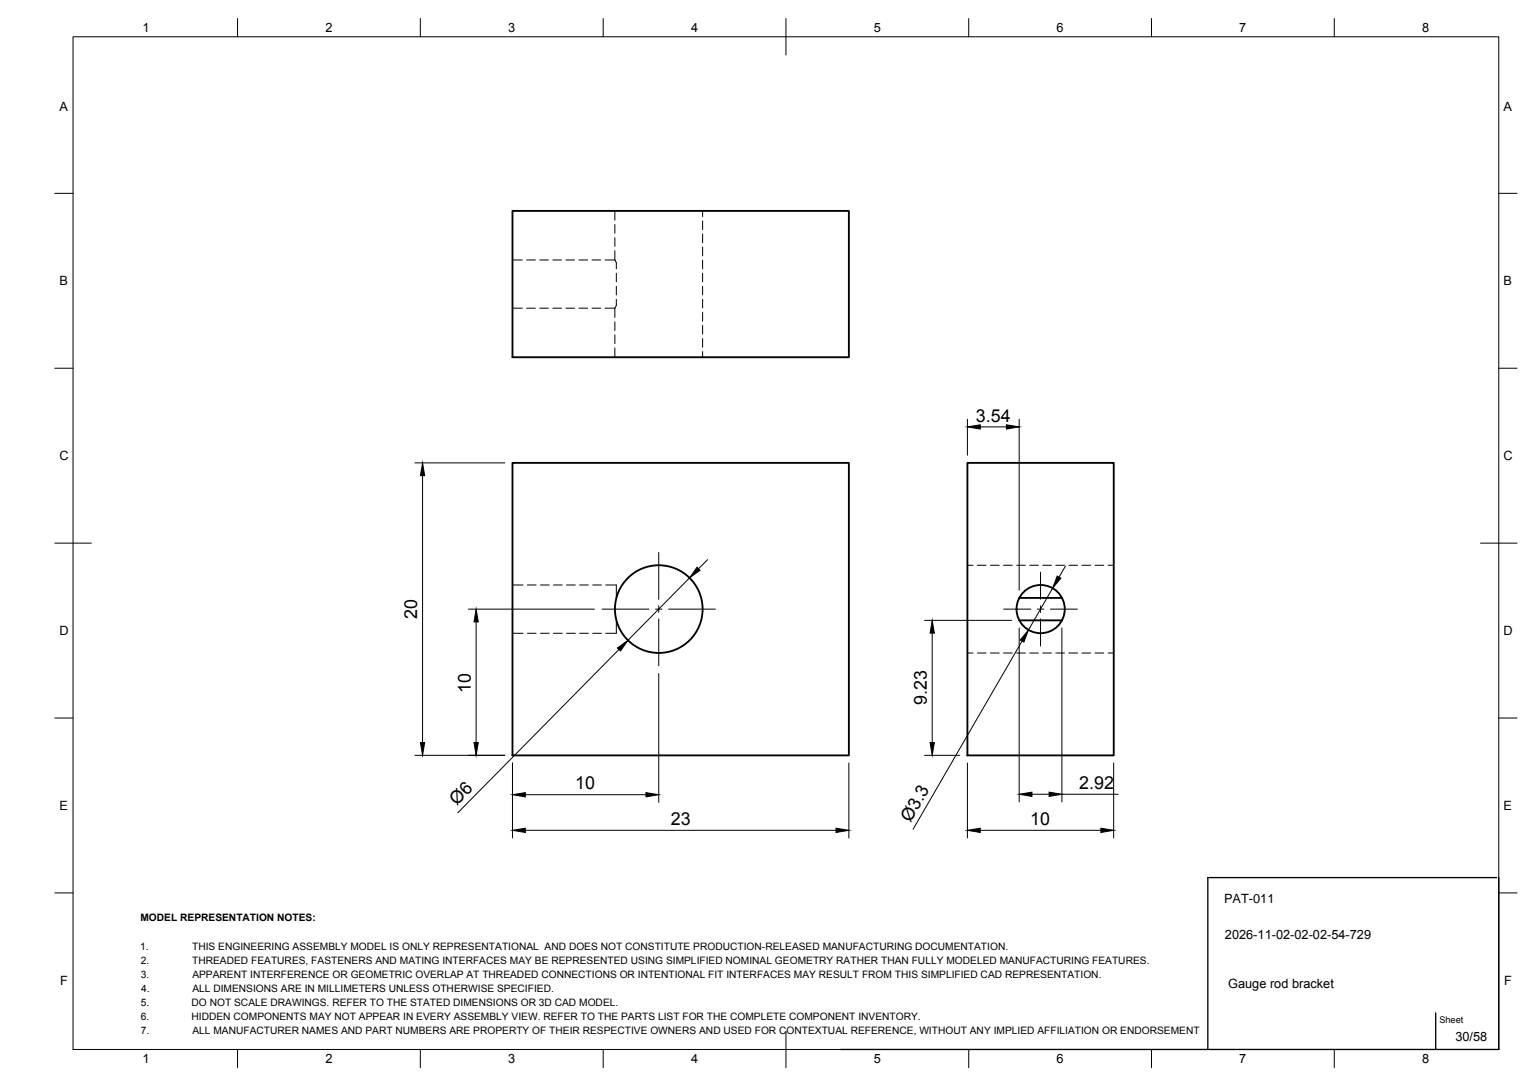
ISO-10303-21;
HEADER;
/* Generated by software containing ST-Developer
 * from STEP Tools, Inc. (www.steptools.com) 
 */

FILE_DESCRIPTION(
/* description */ ('Belt tension measurement rig'),
/* implementation_level */ '2;1');

FILE_NAME(
/* name */ 'Gauge rod bracket.step',
/* time_stamp */ '2026-10-28T03:24:44-07:00',
/* author */ (''),
/* organization */ (''),
/* preprocessor_version */ 'ST-DEVELOPER v20.2',
/* originating_system */ 'Autodesk Translation Framework v15.17.0.0',
/* authorisation */ '');

FILE_SCHEMA (('AUTOMOTIVE_DESIGN { 1 0 10303 214 3 1 1 }'));
ENDSEC;

DATA;
#10=MECHANICAL_DESIGN_GEOMETRIC_PRESENTATION_REPRESENTATION('',(#726),#23587);
#513=B_SPLINE_CURVE_WITH_KNOTS('',3,(#20469,#20470,#20471,#20472,#20473,
#20474),.UNSPECIFIED.,.F.,.F.,(4,2,4),(0.687371506923446,0.701311490231616,
0.764919212052549),.UNSPECIFIED.);
#514=B_SPLINE_CURVE_WITH_KNOTS('',3,(#20478,#20479,#20480,#20481,#20482,
#20483),.UNSPECIFIED.,.F.,.F.,(4,2,4),(0.254973070684183,0.318580792505116,
0.332520775813288),.UNSPECIFIED.);
#515=B_SPLINE_CURVE_WITH_KNOTS('',3,(#20484,#20485,#20486,#20487,#20488,
#20489),.UNSPECIFIED.,.F.,.F.,(4,2,4),(0.177425365555078,0.19136534886325,
0.254973070684183),.UNSPECIFIED.);
#516=B_SPLINE_CURVE_WITH_KNOTS('',3,(#20490,#20491,#20492,#20493,#20494,
#20495),.UNSPECIFIED.,.F.,.F.,(4,2,4),(0.764919212052549,0.828526933873482,
0.842466917181652),.UNSPECIFIED.);
#608=SHAPE_REPRESENTATION_RELATIONSHIP('SRR','None',#23855,#663);
#663=ADVANCED_BREP_SHAPE_REPRESENTATION('',(#796),#23553);
#726=STYLED_ITEM('',(#24211),#796);
#796=MANIFOLD_SOLID_BREP('Body1',#12231);
#966=FACE_BOUND('',#2514,.T.);
#967=FACE_BOUND('',#2517,.T.);
#968=FACE_BOUND('',#2519,.T.);
#1193=PLANE('',#13549);
#1194=PLANE('',#13554);
#1195=PLANE('',#13558);
#1196=PLANE('',#13559);
#1197=PLANE('',#13560);
#1198=PLANE('',#13561);
#1199=PLANE('',#13562);
#1200=PLANE('',#13563);
#1667=FACE_OUTER_BOUND('',#2508,.T.);
#1668=FACE_OUTER_BOUND('',#2509,.T.);
#1669=FACE_OUTER_BOUND('',#2510,.T.);
#1670=FACE_OUTER_BOUND('',#2511,.T.);
#1671=FACE_OUTER_BOUND('',#2512,.T.);
#1672=FACE_OUTER_BOUND('',#2513,.T.);
#1673=FACE_OUTER_BOUND('',#2515,.T.);
#1674=FACE_OUTER_BOUND('',#2516,.T.);
#1675=FACE_OUTER_BOUND('',#2518,.T.);
#1676=FACE_OUTER_BOUND('',#2520,.T.);
#2508=EDGE_LOOP('',(#9310,#9311));
#2509=EDGE_LOOP('',(#9312,#9313,#9314,#9315,#9316,#9317,#9318,#9319,#9320));
#2510=EDGE_LOOP('',(#9321,#9322));
#2511=EDGE_LOOP('',(#9323,#9324,#9325,#9326,#9327,#9328,#9329,#9330,#9331,
#9332,#9333,#9334));
#2512=EDGE_LOOP('',(#9335,#9336,#9337,#9338));
#2513=EDGE_LOOP('',(#9339,#9340,#9341,#9342));
#2514=EDGE_LOOP('',(#9343));
#2515=EDGE_LOOP('',(#9344,#9345,#9346,#9347));
#2516=EDGE_LOOP('',(#9348,#9349,#9350,#9351));
#2517=EDGE_LOOP('',(#9352));
#2518=EDGE_LOOP('',(#9353,#9354,#9355,#9356));
#2519=EDGE_LOOP('',(#9357));
#2520=EDGE_LOOP('',(#9358,#9359,#9360,#9361));
#3310=LINE('',#20464,#4061);
#3311=LINE('',#20497,#4062);
#3312=LINE('',#20500,#4063);
#3313=LINE('',#20504,#4064);
#3314=LINE('',#20506,#4065);
#3315=LINE('',#20511,#4066);
#3316=LINE('',#20513,#4067);
#3317=LINE('',#20515,#4068);
#3318=LINE('',#20516,#4069);
#3319=LINE('',#20519,#4070);
#3320=LINE('',#20521,#4071);
#3321=LINE('',#20522,#4072);
#3322=LINE('',#20525,#4073);
#3323=LINE('',#20527,#4074);
#3324=LINE('',#20528,#4075);
#3325=LINE('',#20530,#4076);
#3326=LINE('',#20531,#4077);
#4061=VECTOR('',#16207,1.);
#4062=VECTOR('',#16214,0.164999999999999);
#4063=VECTOR('',#16219,1.);
#4064=VECTOR('',#16224,0.3);
#4065=VECTOR('',#16225,0.3);
#4066=VECTOR('',#16230,1.);
#4067=VECTOR('',#16231,1.);
#4068=VECTOR('',#16232,1.);
#4069=VECTOR('',#16233,1.);
#4070=VECTOR('',#16236,1.);
#4071=VECTOR('',#16237,1.);
#4072=VECTOR('',#16238,1.);
#4073=VECTOR('',#16241,1.);
#4074=VECTOR('',#16242,1.);
#4075=VECTOR('',#16243,1.);
#4076=VECTOR('',#16246,1.);
#4077=VECTOR('',#16247,1.);
#4792=CIRCLE('',#13550,0.164999999999999);
#4793=CIRCLE('',#13552,0.164999999999999);
#4794=CIRCLE('',#13553,0.164999999999999);
#4795=CIRCLE('',#13556,0.3);
#4796=CIRCLE('',#13557,0.3);
#5702=VERTEX_POINT('',#20462);
#5703=VERTEX_POINT('',#20463);
#5704=VERTEX_POINT('',#20467);
#5705=VERTEX_POINT('',#20468);
#5706=VERTEX_POINT('',#20475);
#5707=VERTEX_POINT('',#20477);
#5708=VERTEX_POINT('',#20496);
#5709=VERTEX_POINT('',#20502);
#5710=VERTEX_POINT('',#20505);
#5711=VERTEX_POINT('',#20509);
#5712=VERTEX_POINT('',#20510);
#5713=VERTEX_POINT('',#20512);
#5714=VERTEX_POINT('',#20514);
#5715=VERTEX_POINT('',#20518);
#5716=VERTEX_POINT('',#20520);
#5717=VERTEX_POINT('',#20524);
#5718=VERTEX_POINT('',#20526);
#7014=EDGE_CURVE('',#5702,#5703,#3310,.T.);
#7015=EDGE_CURVE('',#5702,#5703,#4792,.T.);
#7016=EDGE_CURVE('',#5704,#5705,#513,.T.);
#7017=EDGE_CURVE('',#5706,#5704,#4793,.T.);
#7018=EDGE_CURVE('',#5707,#5706,#514,.T.);
#7019=EDGE_CURVE('',#5703,#5707,#515,.T.);
#7020=EDGE_CURVE('',#5705,#5702,#516,.T.);
#7021=EDGE_CURVE('',#5705,#5708,#3311,.T.);
#7022=EDGE_CURVE('',#5708,#5708,#4794,.T.);
#7023=EDGE_CURVE('',#5706,#5704,#3312,.T.);
#7024=EDGE_CURVE('',#5709,#5709,#4795,.T.);
#7025=EDGE_CURVE('',#5709,#5705,#3313,.T.);
#7026=EDGE_CURVE('',#5707,#5710,#3314,.T.);
#7027=EDGE_CURVE('',#5710,#5710,#4796,.T.);
#7028=EDGE_CURVE('',#5711,#5712,#3315,.T.);
#7029=EDGE_CURVE('',#5712,#5713,#3316,.T.);
#7030=EDGE_CURVE('',#5714,#5713,#3317,.T.);
#7031=EDGE_CURVE('',#5711,#5714,#3318,.T.);
#7032=EDGE_CURVE('',#5715,#5711,#3319,.T.);
#7033=EDGE_CURVE('',#5716,#5714,#3320,.T.);
#7034=EDGE_CURVE('',#5715,#5716,#3321,.T.);
#7035=EDGE_CURVE('',#5717,#5715,#3322,.T.);
#7036=EDGE_CURVE('',#5718,#5716,#3323,.T.);
#7037=EDGE_CURVE('',#5717,#5718,#3324,.T.);
#7038=EDGE_CURVE('',#5712,#5717,#3325,.T.);
#7039=EDGE_CURVE('',#5713,#5718,#3326,.T.);
#9310=ORIENTED_EDGE('',*,*,#7014,.F.);
#9311=ORIENTED_EDGE('',*,*,#7015,.T.);
#9312=ORIENTED_EDGE('',*,*,#7016,.F.);
#9313=ORIENTED_EDGE('',*,*,#7017,.F.);
#9314=ORIENTED_EDGE('',*,*,#7018,.F.);
#9315=ORIENTED_EDGE('',*,*,#7019,.F.);
#9316=ORIENTED_EDGE('',*,*,#7015,.F.);
#9317=ORIENTED_EDGE('',*,*,#7020,.F.);
#9318=ORIENTED_EDGE('',*,*,#7021,.T.);
#9319=ORIENTED_EDGE('',*,*,#7022,.F.);
#9320=ORIENTED_EDGE('',*,*,#7021,.F.);
#9321=ORIENTED_EDGE('',*,*,#7023,.F.);
#9322=ORIENTED_EDGE('',*,*,#7017,.T.);
#9323=ORIENTED_EDGE('',*,*,#7024,.F.);
#9324=ORIENTED_EDGE('',*,*,#7025,.T.);
#9325=ORIENTED_EDGE('',*,*,#7020,.T.);
#9326=ORIENTED_EDGE('',*,*,#7014,.T.);
#9327=ORIENTED_EDGE('',*,*,#7019,.T.);
#9328=ORIENTED_EDGE('',*,*,#7026,.T.);
#9329=ORIENTED_EDGE('',*,*,#7027,.F.);
#9330=ORIENTED_EDGE('',*,*,#7026,.F.);
#9331=ORIENTED_EDGE('',*,*,#7018,.T.);
#9332=ORIENTED_EDGE('',*,*,#7023,.T.);
#9333=ORIENTED_EDGE('',*,*,#7016,.T.);
#9334=ORIENTED_EDGE('',*,*,#7025,.F.);
#9335=ORIENTED_EDGE('',*,*,#7028,.T.);
#9336=ORIENTED_EDGE('',*,*,#7029,.T.);
#9337=ORIENTED_EDGE('',*,*,#7030,.F.);
#9338=ORIENTED_EDGE('',*,*,#7031,.F.);
#9339=ORIENTED_EDGE('',*,*,#7032,.T.);
#9340=ORIENTED_EDGE('',*,*,#7031,.T.);
#9341=ORIENTED_EDGE('',*,*,#7033,.F.);
#9342=ORIENTED_EDGE('',*,*,#7034,.F.);
#9343=ORIENTED_EDGE('',*,*,#7027,.T.);
#9344=ORIENTED_EDGE('',*,*,#7035,.T.);
#9345=ORIENTED_EDGE('',*,*,#7034,.T.);
#9346=ORIENTED_EDGE('',*,*,#7036,.F.);
#9347=ORIENTED_EDGE('',*,*,#7037,.F.);
#9348=ORIENTED_EDGE('',*,*,#7038,.T.);
#9349=ORIENTED_EDGE('',*,*,#7037,.T.);
#9350=ORIENTED_EDGE('',*,*,#7039,.F.);
#9351=ORIENTED_EDGE('',*,*,#7029,.F.);
#9352=ORIENTED_EDGE('',*,*,#7024,.T.);
#9353=ORIENTED_EDGE('',*,*,#7039,.T.);
#9354=ORIENTED_EDGE('',*,*,#7036,.T.);
#9355=ORIENTED_EDGE('',*,*,#7033,.T.);
#9356=ORIENTED_EDGE('',*,*,#7030,.T.);
#9357=ORIENTED_EDGE('',*,*,#7022,.T.);
#9358=ORIENTED_EDGE('',*,*,#7038,.F.);
#9359=ORIENTED_EDGE('',*,*,#7028,.F.);
#9360=ORIENTED_EDGE('',*,*,#7032,.F.);
#9361=ORIENTED_EDGE('',*,*,#7035,.F.);
#11295=CYLINDRICAL_SURFACE('',#13551,0.164999999999999);
#11296=CYLINDRICAL_SURFACE('',#13555,0.3);
#11808=ADVANCED_FACE('',(#1667),#1193,.T.);
#11809=ADVANCED_FACE('',(#1668),#11295,.F.);
#11810=ADVANCED_FACE('',(#1669),#1194,.T.);
#11811=ADVANCED_FACE('',(#1670),#11296,.F.);
#11812=ADVANCED_FACE('',(#1671),#1195,.T.);
#11813=ADVANCED_FACE('',(#1672,#966),#1196,.T.);
#11814=ADVANCED_FACE('',(#1673),#1197,.T.);
#11815=ADVANCED_FACE('',(#1674,#967),#1198,.T.);
#11816=ADVANCED_FACE('',(#1675,#968),#1199,.T.);
#11817=ADVANCED_FACE('',(#1676),#1200,.F.);
#12231=CLOSED_SHELL('',(#11808,#11809,#11810,#11811,#11812,#11813,#11814,
#11815,#11816,#11817));
#13548=AXIS2_PLACEMENT_3D('',#20460,#16203,#16204);
#13549=AXIS2_PLACEMENT_3D('',#20461,#16205,#16206);
#13550=AXIS2_PLACEMENT_3D('',#20465,#16208,#16209);
#13551=AXIS2_PLACEMENT_3D('',#20466,#16210,#16211);
#13552=AXIS2_PLACEMENT_3D('',#20476,#16212,#16213);
#13553=AXIS2_PLACEMENT_3D('',#20498,#16215,#16216);
#13554=AXIS2_PLACEMENT_3D('',#20499,#16217,#16218);
#13555=AXIS2_PLACEMENT_3D('',#20501,#16220,#16221);
#13556=AXIS2_PLACEMENT_3D('',#20503,#16222,#16223);
#13557=AXIS2_PLACEMENT_3D('',#20507,#16226,#16227);
#13558=AXIS2_PLACEMENT_3D('',#20508,#16228,#16229);
#13559=AXIS2_PLACEMENT_3D('',#20517,#16234,#16235);
#13560=AXIS2_PLACEMENT_3D('',#20523,#16239,#16240);
#13561=AXIS2_PLACEMENT_3D('',#20529,#16244,#16245);
#13562=AXIS2_PLACEMENT_3D('',#20532,#16248,#16249);
#13563=AXIS2_PLACEMENT_3D('',#20533,#16250,#16251);
#16203=DIRECTION('axis',(0.,0.,1.));
#16204=DIRECTION('refdir',(1.,0.,0.));
#16205=DIRECTION('center_axis',(0.,0.,1.));
#16206=DIRECTION('ref_axis',(1.,0.,0.));
#16207=DIRECTION('',(1.,0.,0.));
#16208=DIRECTION('center_axis',(0.,0.,1.));
#16209=DIRECTION('ref_axis',(1.,0.,0.));
#16210=DIRECTION('center_axis',(0.,0.,1.));
#16211=DIRECTION('ref_axis',(1.,0.,0.));
#16212=DIRECTION('center_axis',(0.,0.,1.));
#16213=DIRECTION('ref_axis',(1.,0.,0.));
#16214=DIRECTION('',(0.,0.,1.));
#16215=DIRECTION('center_axis',(0.,0.,-1.));
#16216=DIRECTION('ref_axis',(1.,0.,0.));
#16217=DIRECTION('center_axis',(0.,0.,1.));
#16218=DIRECTION('ref_axis',(1.,0.,0.));
#16219=DIRECTION('',(-1.,0.,0.));
#16220=DIRECTION('center_axis',(1.,0.,0.));
#16221=DIRECTION('ref_axis',(0.,0.,-1.));
#16222=DIRECTION('center_axis',(1.,0.,0.));
#16223=DIRECTION('ref_axis',(0.,0.,-1.));
#16224=DIRECTION('',(1.,0.,0.));
#16225=DIRECTION('',(1.,0.,0.));
#16226=DIRECTION('center_axis',(-1.,0.,0.));
#16227=DIRECTION('ref_axis',(0.,0.,-1.));
#16228=DIRECTION('center_axis',(0.,1.,0.));
#16229=DIRECTION('ref_axis',(-1.,0.,0.));
#16230=DIRECTION('',(-1.,0.,0.));
#16231=DIRECTION('',(0.,0.,1.));
#16232=DIRECTION('',(-1.,0.,0.));
#16233=DIRECTION('',(0.,0.,1.));
#16234=DIRECTION('center_axis',(1.,0.,0.));
#16235=DIRECTION('ref_axis',(0.,1.,0.));
#16236=DIRECTION('',(0.,1.,0.));
#16237=DIRECTION('',(0.,1.,0.));
#16238=DIRECTION('',(0.,0.,1.));
#16239=DIRECTION('center_axis',(0.,-1.,0.));
#16240=DIRECTION('ref_axis',(1.,0.,0.));
#16241=DIRECTION('',(1.,0.,0.));
#16242=DIRECTION('',(1.,0.,0.));
#16243=DIRECTION('',(0.,0.,1.));
#16244=DIRECTION('center_axis',(-1.,0.,0.));
#16245=DIRECTION('ref_axis',(0.,-1.,0.));
#16246=DIRECTION('',(0.,-1.,0.));
#16247=DIRECTION('',(0.,-1.,0.));
#16248=DIRECTION('center_axis',(0.,0.,1.));
#16249=DIRECTION('ref_axis',(1.,0.,0.));
#16250=DIRECTION('center_axis',(0.,0.,1.));
#16251=DIRECTION('ref_axis',(1.,0.,0.));
#20460=CARTESIAN_POINT('',(0.,0.,0.));
#20461=CARTESIAN_POINT('Origin',(13.5,7.5,4.79));
#20462=CARTESIAN_POINT('',(13.3539691813349,7.42318854252131,4.79));
#20463=CARTESIAN_POINT('',(13.6460308186651,7.42318854252131,4.79));
#20464=CARTESIAN_POINT('',(12.9,7.42318854252131,4.79));
#20465=CARTESIAN_POINT('Origin',(13.5,7.5,4.79));
#20466=CARTESIAN_POINT('Origin',(13.5,7.5,4.79));
#20467=CARTESIAN_POINT('',(13.3539691813349,7.57681145747869,4.79));
#20468=CARTESIAN_POINT('',(13.335,7.5,4.8));
#20469=CARTESIAN_POINT('Ctrl Pts',(13.3539691813349,7.57681145747868,4.79));
#20470=CARTESIAN_POINT('Ctrl Pts',(13.3517424038809,7.57257799875687,4.79112130391241));
#20471=CARTESIAN_POINT('Ctrl Pts',(13.3496896532208,7.56822754447862,4.79217403693718));
#20472=CARTESIAN_POINT('Ctrl Pts',(13.3393317115009,7.54351674734392,4.79755094970157));
#20473=CARTESIAN_POINT('Ctrl Pts',(13.335,7.52120257394031,4.8));
#20474=CARTESIAN_POINT('Ctrl Pts',(13.335,7.5,4.8));
#20475=CARTESIAN_POINT('',(13.6460308186651,7.57681145747869,4.79));
#20476=CARTESIAN_POINT('Origin',(13.5,7.5,4.79));
#20477=CARTESIAN_POINT('',(13.665,7.5,4.8));
#20478=CARTESIAN_POINT('Ctrl Pts',(13.665,7.5,4.8));
#20479=CARTESIAN_POINT('Ctrl Pts',(13.665,7.52120257394031,4.8));
#20480=CARTESIAN_POINT('Ctrl Pts',(13.6606682884991,7.54351674734392,4.79755094970157));
#20481=CARTESIAN_POINT('Ctrl Pts',(13.6503103467792,7.56822754447862,4.79217403693718));
#20482=CARTESIAN_POINT('Ctrl Pts',(13.6482575961191,7.57257799875688,4.79112130391241));
#20483=CARTESIAN_POINT('Ctrl Pts',(13.6460308186651,7.57681145747869,4.79));
#20484=CARTESIAN_POINT('Ctrl Pts',(13.6460308186651,7.42318854252131,4.79));
#20485=CARTESIAN_POINT('Ctrl Pts',(13.6482575961191,7.42742200124312,4.79112130391241));
#20486=CARTESIAN_POINT('Ctrl Pts',(13.6503103467792,7.43177245552138,4.79217403693718));
#20487=CARTESIAN_POINT('Ctrl Pts',(13.6606682884991,7.45648325265608,4.79755094970157));
#20488=CARTESIAN_POINT('Ctrl Pts',(13.665,7.47879742605969,4.8));
#20489=CARTESIAN_POINT('Ctrl Pts',(13.665,7.5,4.8));
#20490=CARTESIAN_POINT('Ctrl Pts',(13.335,7.5,4.8));
#20491=CARTESIAN_POINT('Ctrl Pts',(13.335,7.47879742605969,4.8));
#20492=CARTESIAN_POINT('Ctrl Pts',(13.3393317115009,7.45648325265608,4.79755094970157));
#20493=CARTESIAN_POINT('Ctrl Pts',(13.3496896532208,7.43177245552138,4.79217403693718));
#20494=CARTESIAN_POINT('Ctrl Pts',(13.3517424038809,7.42742200124312,4.79112130391241));
#20495=CARTESIAN_POINT('Ctrl Pts',(13.3539691813349,7.42318854252132,4.79));
#20496=CARTESIAN_POINT('',(13.335,7.5,5.5));
#20497=CARTESIAN_POINT('',(13.335,7.5,4.79));
#20498=CARTESIAN_POINT('Origin',(13.5,7.5,5.5));
#20499=CARTESIAN_POINT('Origin',(13.5,7.5,4.79));
#20500=CARTESIAN_POINT('',(12.9,7.57681145747869,4.79));
#20501=CARTESIAN_POINT('Origin',(12.9,7.5,4.5));
#20502=CARTESIAN_POINT('',(13.,7.5,4.8));
#20503=CARTESIAN_POINT('Origin',(13.,7.5,4.5));
#20504=CARTESIAN_POINT('',(12.9,7.5,4.8));
#20505=CARTESIAN_POINT('',(14.,7.5,4.8));
#20506=CARTESIAN_POINT('',(12.9,7.5,4.8));
#20507=CARTESIAN_POINT('Origin',(14.,7.5,4.5));
#20508=CARTESIAN_POINT('Origin',(14.,8.5,3.2));
#20509=CARTESIAN_POINT('',(14.,8.5,3.2));
#20510=CARTESIAN_POINT('',(13.,8.5,3.2));
#20511=CARTESIAN_POINT('',(14.,8.5,3.2));
#20512=CARTESIAN_POINT('',(13.,8.5,5.5));
#20513=CARTESIAN_POINT('',(13.,8.5,3.2));
#20514=CARTESIAN_POINT('',(14.,8.5,5.5));
#20515=CARTESIAN_POINT('',(14.,8.5,5.5));
#20516=CARTESIAN_POINT('',(14.,8.5,3.2));
#20517=CARTESIAN_POINT('Origin',(14.,6.5,3.2));
#20518=CARTESIAN_POINT('',(14.,6.5,3.2));
#20519=CARTESIAN_POINT('',(14.,6.5,3.2));
#20520=CARTESIAN_POINT('',(14.,6.5,5.5));
#20521=CARTESIAN_POINT('',(14.,6.5,5.5));
#20522=CARTESIAN_POINT('',(14.,6.5,3.2));
#20523=CARTESIAN_POINT('Origin',(13.,6.5,3.2));
#20524=CARTESIAN_POINT('',(13.,6.5,3.2));
#20525=CARTESIAN_POINT('',(13.,6.5,3.2));
#20526=CARTESIAN_POINT('',(13.,6.5,5.5));
#20527=CARTESIAN_POINT('',(13.,6.5,5.5));
#20528=CARTESIAN_POINT('',(13.,6.5,3.2));
#20529=CARTESIAN_POINT('Origin',(13.,8.5,3.2));
#20530=CARTESIAN_POINT('',(13.,8.5,3.2));
#20531=CARTESIAN_POINT('',(13.,8.5,5.5));
#20532=CARTESIAN_POINT('Origin',(13.5,7.5,5.5));
#20533=CARTESIAN_POINT('Origin',(13.5,7.5,3.2));
#23488=UNCERTAINTY_MEASURE_WITH_UNIT(LENGTH_MEASURE(0.001),#23588,
'DISTANCE_ACCURACY_VALUE',
'Maximum model space distance between geometric entities at asserted c
onnectivities');
#23522=UNCERTAINTY_MEASURE_WITH_UNIT(LENGTH_MEASURE(0.001),#23588,
'DISTANCE_ACCURACY_VALUE',
'Maximum model space distance between geometric entities at asserted c
onnectivities');
#23553=(
GEOMETRIC_REPRESENTATION_CONTEXT(3)
GLOBAL_UNCERTAINTY_ASSIGNED_CONTEXT((#23488))
GLOBAL_UNIT_ASSIGNED_CONTEXT((#23588,#23590,#23591))
REPRESENTATION_CONTEXT('','3D')
);
#23587=(
GEOMETRIC_REPRESENTATION_CONTEXT(3)
GLOBAL_UNCERTAINTY_ASSIGNED_CONTEXT((#23522))
GLOBAL_UNIT_ASSIGNED_CONTEXT((#23588,#23590,#23591))
REPRESENTATION_CONTEXT('','3D')
);
#23588=(
LENGTH_UNIT()
NAMED_UNIT(*)
SI_UNIT(.CENTI.,.METRE.)
);
#23590=(
NAMED_UNIT(*)
PLANE_ANGLE_UNIT()
SI_UNIT($,.RADIAN.)
);
#23591=(
NAMED_UNIT(*)
SI_UNIT($,.STERADIAN.)
SOLID_ANGLE_UNIT()
);
#23622=SHAPE_DEFINITION_REPRESENTATION(#23691,#23855);
#23691=PRODUCT_DEFINITION_SHAPE('',$,#23920);
#23855=SHAPE_REPRESENTATION('',(#13548),#23553);
#23889=PRODUCT_DEFINITION_CONTEXT('part definition',#24083,'design');
#23920=PRODUCT_DEFINITION('Gauge rod bracket','Gauge rod bracket',#23984,
#23889);
#23984=PRODUCT_DEFINITION_FORMATION('',$,#24115);
#24083=APPLICATION_CONTEXT(
'Core Data for Automotive Mechanical Design Process');
#24084=PRODUCT_CONTEXT('part definition',#24083,'mechanical');
#24115=PRODUCT('Gauge rod bracket','Gauge rod bracket',
'Gauge rod bracket',(#24084));
#24205=COLOUR_RGB('Grey',0.48,0.52,0.57);
#24206=FILL_AREA_STYLE_COLOUR('',#24205);
#24207=FILL_AREA_STYLE('',(#24206));
#24208=SURFACE_STYLE_FILL_AREA(#24207);
#24209=SURFACE_SIDE_STYLE('',(#24208));
#24210=SURFACE_STYLE_USAGE(.BOTH.,#24209);
#24211=PRESENTATION_STYLE_ASSIGNMENT((#24210));
ENDSEC;
END-ISO-10303-21;
